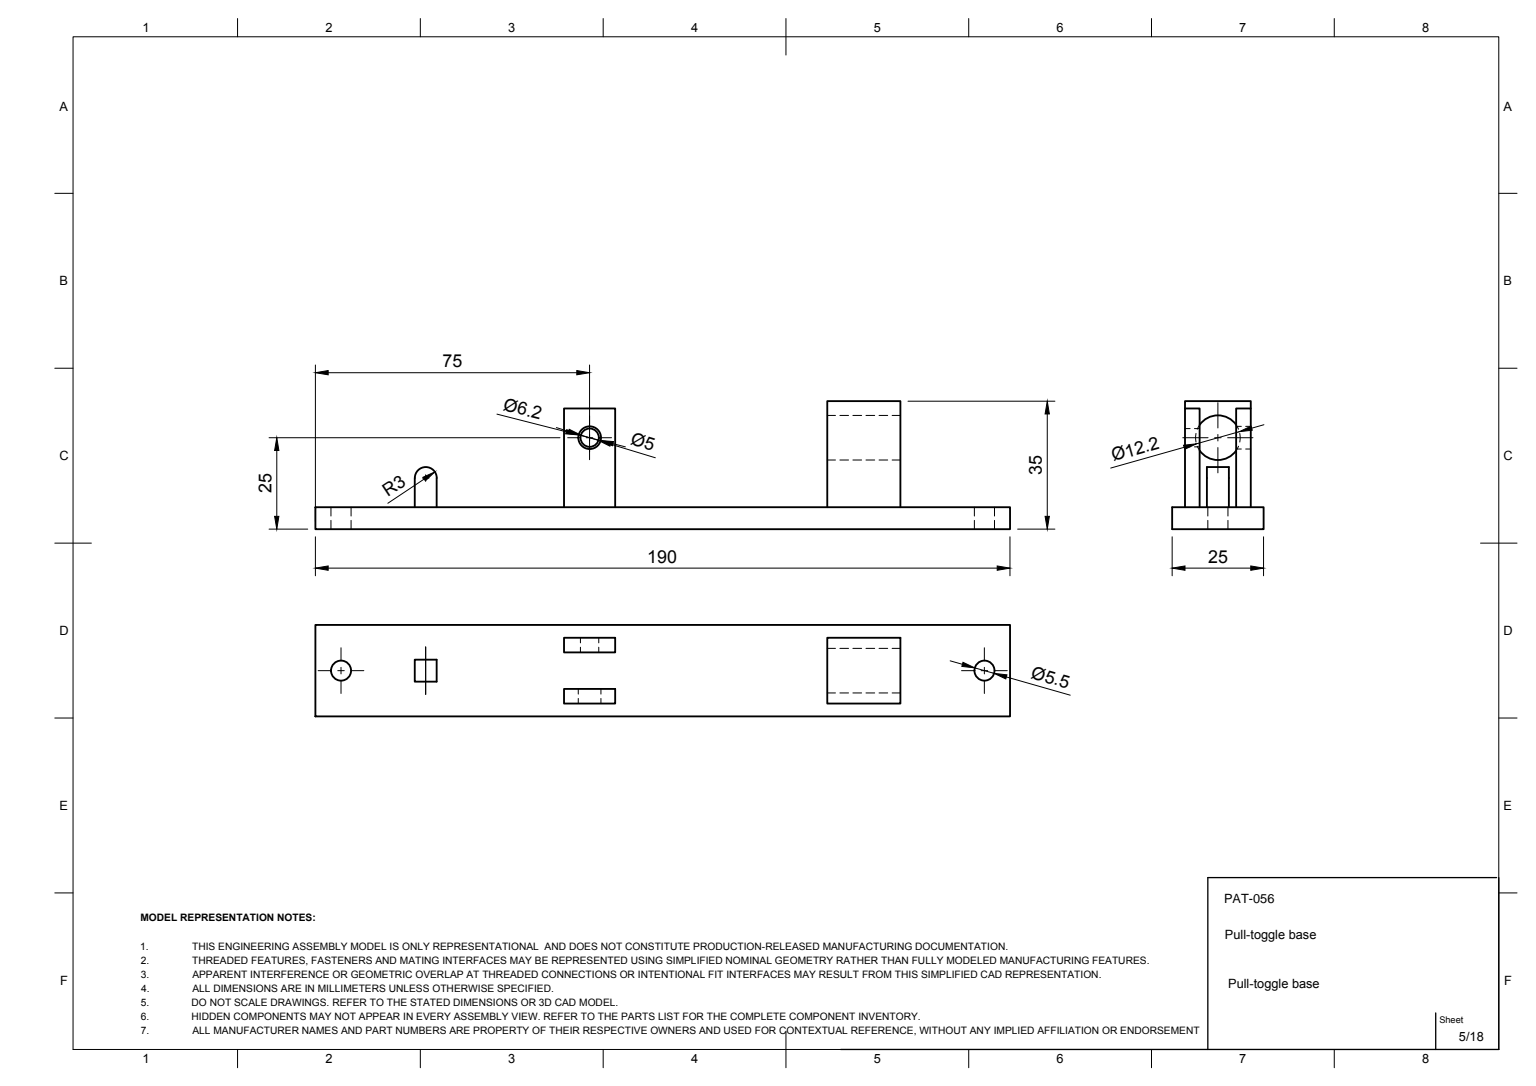
ISO-10303-21;
HEADER;
/* Generated by software containing ST-Developer
 * from STEP Tools, Inc. (www.steptools.com) 
 */

FILE_DESCRIPTION(
/* description */ ('Hook toggle clamp'),
/* implementation_level */ '2;1');

FILE_NAME(
/* name */ 'Pull-toggle base.step',
/* time_stamp */ '2026-10-27T21:56:56-07:00',
/* author */ (''),
/* organization */ (''),
/* preprocessor_version */ 'ST-DEVELOPER v20.2',
/* originating_system */ 'Autodesk Translation Framework v15.17.0.0',
/* authorisation */ '');

FILE_SCHEMA (('AUTOMOTIVE_DESIGN { 1 0 10303 214 3 1 1 }'));
ENDSEC;

DATA;
#10=MECHANICAL_DESIGN_GEOMETRIC_PRESENTATION_REPRESENTATION('',(#189),#5458);
#155=SHAPE_REPRESENTATION_RELATIONSHIP('SRR','None',#5536,#172);
#172=ADVANCED_BREP_SHAPE_REPRESENTATION('',(#206),#5438);
#189=STYLED_ITEM('',(#5696),#206);
#206=MANIFOLD_SOLID_BREP('Body1',#2970);
#222=FACE_BOUND('',#577,.T.);
#223=FACE_BOUND('',#579,.T.);
#224=FACE_BOUND('',#584,.T.);
#225=FACE_BOUND('',#589,.T.);
#226=FACE_BOUND('',#591,.T.);
#227=FACE_BOUND('',#596,.T.);
#228=FACE_BOUND('',#602,.T.);
#229=FACE_BOUND('',#603,.T.);
#230=FACE_BOUND('',#604,.T.);
#231=FACE_BOUND('',#605,.T.);
#232=FACE_BOUND('',#606,.T.);
#233=FACE_BOUND('',#607,.T.);
#234=FACE_BOUND('',#609,.T.);
#235=FACE_BOUND('',#610,.T.);
#278=PLANE('',#3182);
#279=PLANE('',#3183);
#280=PLANE('',#3184);
#281=PLANE('',#3188);
#282=PLANE('',#3198);
#283=PLANE('',#3199);
#284=PLANE('',#3200);
#285=PLANE('',#3201);
#286=PLANE('',#3202);
#287=PLANE('',#3206);
#288=PLANE('',#3207);
#289=PLANE('',#3208);
#290=PLANE('',#3209);
#291=PLANE('',#3210);
#292=PLANE('',#3211);
#293=PLANE('',#3212);
#294=PLANE('',#3213);
#295=PLANE('',#3214);
#296=PLANE('',#3215);
#297=PLANE('',#3216);
#298=PLANE('',#3217);
#299=PLANE('',#3218);
#300=PLANE('',#3219);
#301=PLANE('',#3220);
#302=PLANE('',#3221);
#393=FACE_OUTER_BOUND('',#566,.T.);
#394=FACE_OUTER_BOUND('',#567,.T.);
#395=FACE_OUTER_BOUND('',#568,.T.);
#396=FACE_OUTER_BOUND('',#569,.T.);
#397=FACE_OUTER_BOUND('',#570,.T.);
#398=FACE_OUTER_BOUND('',#571,.T.);
#399=FACE_OUTER_BOUND('',#572,.T.);
#400=FACE_OUTER_BOUND('',#573,.T.);
#401=FACE_OUTER_BOUND('',#574,.T.);
#402=FACE_OUTER_BOUND('',#575,.T.);
#403=FACE_OUTER_BOUND('',#576,.T.);
#404=FACE_OUTER_BOUND('',#578,.T.);
#405=FACE_OUTER_BOUND('',#580,.T.);
#406=FACE_OUTER_BOUND('',#581,.T.);
#407=FACE_OUTER_BOUND('',#582,.T.);
#408=FACE_OUTER_BOUND('',#583,.T.);
#409=FACE_OUTER_BOUND('',#585,.T.);
#410=FACE_OUTER_BOUND('',#586,.T.);
#411=FACE_OUTER_BOUND('',#587,.T.);
#412=FACE_OUTER_BOUND('',#588,.T.);
#413=FACE_OUTER_BOUND('',#590,.T.);
#414=FACE_OUTER_BOUND('',#592,.T.);
#415=FACE_OUTER_BOUND('',#593,.T.);
#416=FACE_OUTER_BOUND('',#594,.T.);
#417=FACE_OUTER_BOUND('',#595,.T.);
#418=FACE_OUTER_BOUND('',#597,.T.);
#419=FACE_OUTER_BOUND('',#598,.T.);
#420=FACE_OUTER_BOUND('',#599,.T.);
#421=FACE_OUTER_BOUND('',#600,.T.);
#422=FACE_OUTER_BOUND('',#601,.T.);
#423=FACE_OUTER_BOUND('',#608,.T.);
#566=EDGE_LOOP('',(#2001,#2002,#2003,#2004));
#567=EDGE_LOOP('',(#2005,#2006,#2007,#2008));
#568=EDGE_LOOP('',(#2009,#2010,#2011,#2012));
#569=EDGE_LOOP('',(#2013,#2014,#2015,#2016));
#570=EDGE_LOOP('',(#2017,#2018,#2019,#2020));
#571=EDGE_LOOP('',(#2021,#2022,#2023,#2024));
#572=EDGE_LOOP('',(#2025,#2026,#2027,#2028));
#573=EDGE_LOOP('',(#2029,#2030,#2031,#2032));
#574=EDGE_LOOP('',(#2033,#2034,#2035,#2036));
#575=EDGE_LOOP('',(#2037,#2038,#2039,#2040));
#576=EDGE_LOOP('',(#2041,#2042,#2043,#2044));
#577=EDGE_LOOP('',(#2045));
#578=EDGE_LOOP('',(#2046,#2047,#2048,#2049));
#579=EDGE_LOOP('',(#2050));
#580=EDGE_LOOP('',(#2051,#2052,#2053,#2054));
#581=EDGE_LOOP('',(#2055,#2056,#2057,#2058));
#582=EDGE_LOOP('',(#2059,#2060,#2061,#2062));
#583=EDGE_LOOP('',(#2063,#2064,#2065,#2066));
#584=EDGE_LOOP('',(#2067));
#585=EDGE_LOOP('',(#2068,#2069,#2070,#2071));
#586=EDGE_LOOP('',(#2072,#2073,#2074,#2075));
#587=EDGE_LOOP('',(#2076,#2077,#2078,#2079));
#588=EDGE_LOOP('',(#2080,#2081,#2082,#2083));
#589=EDGE_LOOP('',(#2084));
#590=EDGE_LOOP('',(#2085,#2086,#2087,#2088));
#591=EDGE_LOOP('',(#2089));
#592=EDGE_LOOP('',(#2090,#2091,#2092,#2093));
#593=EDGE_LOOP('',(#2094,#2095,#2096,#2097));
#594=EDGE_LOOP('',(#2098,#2099,#2100,#2101));
#595=EDGE_LOOP('',(#2102,#2103,#2104,#2105));
#596=EDGE_LOOP('',(#2106));
#597=EDGE_LOOP('',(#2107,#2108,#2109,#2110));
#598=EDGE_LOOP('',(#2111,#2112,#2113,#2114));
#599=EDGE_LOOP('',(#2115,#2116,#2117,#2118));
#600=EDGE_LOOP('',(#2119,#2120,#2121,#2122));
#601=EDGE_LOOP('',(#2123,#2124,#2125,#2126));
#602=EDGE_LOOP('',(#2127,#2128,#2129,#2130));
#603=EDGE_LOOP('',(#2131));
#604=EDGE_LOOP('',(#2132));
#605=EDGE_LOOP('',(#2133,#2134,#2135,#2136));
#606=EDGE_LOOP('',(#2137,#2138,#2139,#2140));
#607=EDGE_LOOP('',(#2141,#2142,#2143,#2144));
#608=EDGE_LOOP('',(#2145,#2146,#2147,#2148));
#609=EDGE_LOOP('',(#2149));
#610=EDGE_LOOP('',(#2150));
#795=LINE('',#4425,#1032);
#796=LINE('',#4430,#1033);
#797=LINE('',#4432,#1034);
#798=LINE('',#4434,#1035);
#799=LINE('',#4435,#1036);
#800=LINE('',#4439,#1037);
#801=LINE('',#4441,#1038);
#802=LINE('',#4443,#1039);
#803=LINE('',#4444,#1040);
#804=LINE('',#4447,#1041);
#805=LINE('',#4451,#1042);
#806=LINE('',#4456,#1043);
#807=LINE('',#4462,#1044);
#808=LINE('',#4468,#1045);
#809=LINE('',#4473,#1046);
#810=LINE('',#4475,#1047);
#811=LINE('',#4477,#1048);
#812=LINE('',#4478,#1049);
#813=LINE('',#4481,#1050);
#814=LINE('',#4483,#1051);
#815=LINE('',#4484,#1052);
#816=LINE('',#4487,#1053);
#817=LINE('',#4489,#1054);
#818=LINE('',#4490,#1055);
#819=LINE('',#4492,#1056);
#820=LINE('',#4494,#1057);
#821=LINE('',#4499,#1058);
#822=LINE('',#4504,#1059);
#823=LINE('',#4506,#1060);
#824=LINE('',#4508,#1061);
#825=LINE('',#4509,#1062);
#826=LINE('',#4512,#1063);
#827=LINE('',#4514,#1064);
#828=LINE('',#4515,#1065);
#829=LINE('',#4518,#1066);
#830=LINE('',#4520,#1067);
#831=LINE('',#4521,#1068);
#832=LINE('',#4523,#1069);
#833=LINE('',#4525,#1070);
#834=LINE('',#4529,#1071);
#835=LINE('',#4531,#1072);
#836=LINE('',#4533,#1073);
#837=LINE('',#4534,#1074);
#838=LINE('',#4537,#1075);
#839=LINE('',#4539,#1076);
#840=LINE('',#4540,#1077);
#841=LINE('',#4543,#1078);
#842=LINE('',#4545,#1079);
#843=LINE('',#4546,#1080);
#844=LINE('',#4548,#1081);
#845=LINE('',#4550,#1082);
#846=LINE('',#4554,#1083);
#847=LINE('',#4556,#1084);
#848=LINE('',#4558,#1085);
#849=LINE('',#4559,#1086);
#850=LINE('',#4562,#1087);
#851=LINE('',#4564,#1088);
#852=LINE('',#4565,#1089);
#853=LINE('',#4568,#1090);
#854=LINE('',#4570,#1091);
#855=LINE('',#4571,#1092);
#856=LINE('',#4573,#1093);
#857=LINE('',#4574,#1094);
#1032=VECTOR('',#3521,0.25);
#1033=VECTOR('',#3526,1.);
#1034=VECTOR('',#3527,1.);
#1035=VECTOR('',#3528,1.);
#1036=VECTOR('',#3529,1.);
#1037=VECTOR('',#3532,1.);
#1038=VECTOR('',#3533,1.);
#1039=VECTOR('',#3534,1.);
#1040=VECTOR('',#3535,1.);
#1041=VECTOR('',#3540,1.);
#1042=VECTOR('',#3547,1.);
#1043=VECTOR('',#3552,0.275);
#1044=VECTOR('',#3559,0.275);
#1045=VECTOR('',#3566,0.61);
#1046=VECTOR('',#3571,1.);
#1047=VECTOR('',#3572,1.);
#1048=VECTOR('',#3573,1.);
#1049=VECTOR('',#3574,1.);
#1050=VECTOR('',#3577,1.);
#1051=VECTOR('',#3578,1.);
#1052=VECTOR('',#3579,1.);
#1053=VECTOR('',#3582,1.);
#1054=VECTOR('',#3583,1.);
#1055=VECTOR('',#3584,1.);
#1056=VECTOR('',#3587,1.);
#1057=VECTOR('',#3590,1.);
#1058=VECTOR('',#3595,0.31);
#1059=VECTOR('',#3600,1.);
#1060=VECTOR('',#3601,1.);
#1061=VECTOR('',#3602,1.);
#1062=VECTOR('',#3603,1.);
#1063=VECTOR('',#3606,1.);
#1064=VECTOR('',#3607,1.);
#1065=VECTOR('',#3608,1.);
#1066=VECTOR('',#3611,1.);
#1067=VECTOR('',#3612,1.);
#1068=VECTOR('',#3613,1.);
#1069=VECTOR('',#3616,1.);
#1070=VECTOR('',#3619,1.);
#1071=VECTOR('',#3622,1.);
#1072=VECTOR('',#3623,1.);
#1073=VECTOR('',#3624,1.);
#1074=VECTOR('',#3625,1.);
#1075=VECTOR('',#3628,1.);
#1076=VECTOR('',#3629,1.);
#1077=VECTOR('',#3630,1.);
#1078=VECTOR('',#3633,1.);
#1079=VECTOR('',#3634,1.);
#1080=VECTOR('',#3635,1.);
#1081=VECTOR('',#3638,1.);
#1082=VECTOR('',#3641,1.);
#1083=VECTOR('',#3644,1.);
#1084=VECTOR('',#3645,1.);
#1085=VECTOR('',#3646,1.);
#1086=VECTOR('',#3647,1.);
#1087=VECTOR('',#3650,1.);
#1088=VECTOR('',#3651,1.);
#1089=VECTOR('',#3652,1.);
#1090=VECTOR('',#3655,1.);
#1091=VECTOR('',#3656,1.);
#1092=VECTOR('',#3657,1.);
#1093=VECTOR('',#3660,1.);
#1094=VECTOR('',#3661,1.);
#1269=CIRCLE('',#3180,0.25);
#1270=CIRCLE('',#3181,0.25);
#1271=CIRCLE('',#3185,0.3);
#1272=CIRCLE('',#3187,0.3);
#1273=CIRCLE('',#3190,0.275);
#1274=CIRCLE('',#3191,0.275);
#1275=CIRCLE('',#3193,0.275);
#1276=CIRCLE('',#3194,0.275);
#1277=CIRCLE('',#3196,0.61);
#1278=CIRCLE('',#3197,0.61);
#1279=CIRCLE('',#3204,0.31);
#1280=CIRCLE('',#3205,0.31);
#1382=VERTEX_POINT('',#4422);
#1383=VERTEX_POINT('',#4424);
#1384=VERTEX_POINT('',#4428);
#1385=VERTEX_POINT('',#4429);
#1386=VERTEX_POINT('',#4431);
#1387=VERTEX_POINT('',#4433);
#1388=VERTEX_POINT('',#4437);
#1389=VERTEX_POINT('',#4438);
#1390=VERTEX_POINT('',#4440);
#1391=VERTEX_POINT('',#4442);
#1392=VERTEX_POINT('',#4453);
#1393=VERTEX_POINT('',#4455);
#1394=VERTEX_POINT('',#4459);
#1395=VERTEX_POINT('',#4461);
#1396=VERTEX_POINT('',#4465);
#1397=VERTEX_POINT('',#4467);
#1398=VERTEX_POINT('',#4471);
#1399=VERTEX_POINT('',#4472);
#1400=VERTEX_POINT('',#4474);
#1401=VERTEX_POINT('',#4476);
#1402=VERTEX_POINT('',#4480);
#1403=VERTEX_POINT('',#4482);
#1404=VERTEX_POINT('',#4486);
#1405=VERTEX_POINT('',#4488);
#1406=VERTEX_POINT('',#4496);
#1407=VERTEX_POINT('',#4498);
#1408=VERTEX_POINT('',#4502);
#1409=VERTEX_POINT('',#4503);
#1410=VERTEX_POINT('',#4505);
#1411=VERTEX_POINT('',#4507);
#1412=VERTEX_POINT('',#4511);
#1413=VERTEX_POINT('',#4513);
#1414=VERTEX_POINT('',#4517);
#1415=VERTEX_POINT('',#4519);
#1416=VERTEX_POINT('',#4527);
#1417=VERTEX_POINT('',#4528);
#1418=VERTEX_POINT('',#4530);
#1419=VERTEX_POINT('',#4532);
#1420=VERTEX_POINT('',#4536);
#1421=VERTEX_POINT('',#4538);
#1422=VERTEX_POINT('',#4542);
#1423=VERTEX_POINT('',#4544);
#1424=VERTEX_POINT('',#4552);
#1425=VERTEX_POINT('',#4553);
#1426=VERTEX_POINT('',#4555);
#1427=VERTEX_POINT('',#4557);
#1428=VERTEX_POINT('',#4561);
#1429=VERTEX_POINT('',#4563);
#1430=VERTEX_POINT('',#4567);
#1431=VERTEX_POINT('',#4569);
#1627=EDGE_CURVE('',#1382,#1382,#1269,.T.);
#1628=EDGE_CURVE('',#1382,#1383,#795,.T.);
#1629=EDGE_CURVE('',#1383,#1383,#1270,.T.);
#1630=EDGE_CURVE('',#1384,#1385,#796,.T.);
#1631=EDGE_CURVE('',#1386,#1384,#797,.T.);
#1632=EDGE_CURVE('',#1387,#1386,#798,.T.);
#1633=EDGE_CURVE('',#1385,#1387,#799,.T.);
#1634=EDGE_CURVE('',#1388,#1389,#800,.T.);
#1635=EDGE_CURVE('',#1390,#1388,#801,.T.);
#1636=EDGE_CURVE('',#1390,#1391,#802,.T.);
#1637=EDGE_CURVE('',#1389,#1391,#803,.T.);
#1638=EDGE_CURVE('',#1390,#1387,#1271,.T.);
#1639=EDGE_CURVE('',#1385,#1388,#804,.T.);
#1640=EDGE_CURVE('',#1391,#1386,#1272,.T.);
#1641=EDGE_CURVE('',#1389,#1384,#805,.T.);
#1642=EDGE_CURVE('',#1392,#1392,#1273,.T.);
#1643=EDGE_CURVE('',#1392,#1393,#806,.T.);
#1644=EDGE_CURVE('',#1393,#1393,#1274,.T.);
#1645=EDGE_CURVE('',#1394,#1394,#1275,.T.);
#1646=EDGE_CURVE('',#1394,#1395,#807,.T.);
#1647=EDGE_CURVE('',#1395,#1395,#1276,.T.);
#1648=EDGE_CURVE('',#1396,#1396,#1277,.T.);
#1649=EDGE_CURVE('',#1396,#1397,#808,.T.);
#1650=EDGE_CURVE('',#1397,#1397,#1278,.T.);
#1651=EDGE_CURVE('',#1398,#1399,#809,.T.);
#1652=EDGE_CURVE('',#1398,#1400,#810,.T.);
#1653=EDGE_CURVE('',#1400,#1401,#811,.T.);
#1654=EDGE_CURVE('',#1401,#1399,#812,.T.);
#1655=EDGE_CURVE('',#1402,#1398,#813,.T.);
#1656=EDGE_CURVE('',#1403,#1402,#814,.T.);
#1657=EDGE_CURVE('',#1400,#1403,#815,.T.);
#1658=EDGE_CURVE('',#1399,#1404,#816,.T.);
#1659=EDGE_CURVE('',#1401,#1405,#817,.T.);
#1660=EDGE_CURVE('',#1404,#1405,#818,.T.);
#1661=EDGE_CURVE('',#1405,#1403,#819,.T.);
#1662=EDGE_CURVE('',#1404,#1402,#820,.T.);
#1663=EDGE_CURVE('',#1406,#1406,#1279,.T.);
#1664=EDGE_CURVE('',#1406,#1407,#821,.T.);
#1665=EDGE_CURVE('',#1407,#1407,#1280,.T.);
#1666=EDGE_CURVE('',#1408,#1409,#822,.T.);
#1667=EDGE_CURVE('',#1408,#1410,#823,.T.);
#1668=EDGE_CURVE('',#1410,#1411,#824,.T.);
#1669=EDGE_CURVE('',#1411,#1409,#825,.T.);
#1670=EDGE_CURVE('',#1412,#1408,#826,.T.);
#1671=EDGE_CURVE('',#1413,#1412,#827,.T.);
#1672=EDGE_CURVE('',#1410,#1413,#828,.T.);
#1673=EDGE_CURVE('',#1409,#1414,#829,.T.);
#1674=EDGE_CURVE('',#1411,#1415,#830,.T.);
#1675=EDGE_CURVE('',#1414,#1415,#831,.T.);
#1676=EDGE_CURVE('',#1415,#1413,#832,.T.);
#1677=EDGE_CURVE('',#1414,#1412,#833,.T.);
#1678=EDGE_CURVE('',#1416,#1417,#834,.T.);
#1679=EDGE_CURVE('',#1416,#1418,#835,.T.);
#1680=EDGE_CURVE('',#1418,#1419,#836,.T.);
#1681=EDGE_CURVE('',#1419,#1417,#837,.T.);
#1682=EDGE_CURVE('',#1420,#1416,#838,.T.);
#1683=EDGE_CURVE('',#1421,#1420,#839,.T.);
#1684=EDGE_CURVE('',#1418,#1421,#840,.T.);
#1685=EDGE_CURVE('',#1417,#1422,#841,.T.);
#1686=EDGE_CURVE('',#1419,#1423,#842,.T.);
#1687=EDGE_CURVE('',#1422,#1423,#843,.T.);
#1688=EDGE_CURVE('',#1423,#1421,#844,.T.);
#1689=EDGE_CURVE('',#1422,#1420,#845,.T.);
#1690=EDGE_CURVE('',#1424,#1425,#846,.T.);
#1691=EDGE_CURVE('',#1425,#1426,#847,.T.);
#1692=EDGE_CURVE('',#1427,#1426,#848,.T.);
#1693=EDGE_CURVE('',#1424,#1427,#849,.T.);
#1694=EDGE_CURVE('',#1428,#1424,#850,.T.);
#1695=EDGE_CURVE('',#1429,#1427,#851,.T.);
#1696=EDGE_CURVE('',#1428,#1429,#852,.T.);
#1697=EDGE_CURVE('',#1430,#1428,#853,.T.);
#1698=EDGE_CURVE('',#1431,#1429,#854,.T.);
#1699=EDGE_CURVE('',#1430,#1431,#855,.T.);
#1700=EDGE_CURVE('',#1425,#1430,#856,.T.);
#1701=EDGE_CURVE('',#1426,#1431,#857,.T.);
#2001=ORIENTED_EDGE('',*,*,#1627,.F.);
#2002=ORIENTED_EDGE('',*,*,#1628,.T.);
#2003=ORIENTED_EDGE('',*,*,#1629,.T.);
#2004=ORIENTED_EDGE('',*,*,#1628,.F.);
#2005=ORIENTED_EDGE('',*,*,#1630,.F.);
#2006=ORIENTED_EDGE('',*,*,#1631,.F.);
#2007=ORIENTED_EDGE('',*,*,#1632,.F.);
#2008=ORIENTED_EDGE('',*,*,#1633,.F.);
#2009=ORIENTED_EDGE('',*,*,#1634,.F.);
#2010=ORIENTED_EDGE('',*,*,#1635,.F.);
#2011=ORIENTED_EDGE('',*,*,#1636,.T.);
#2012=ORIENTED_EDGE('',*,*,#1637,.F.);
#2013=ORIENTED_EDGE('',*,*,#1638,.F.);
#2014=ORIENTED_EDGE('',*,*,#1635,.T.);
#2015=ORIENTED_EDGE('',*,*,#1639,.F.);
#2016=ORIENTED_EDGE('',*,*,#1633,.T.);
#2017=ORIENTED_EDGE('',*,*,#1636,.F.);
#2018=ORIENTED_EDGE('',*,*,#1638,.T.);
#2019=ORIENTED_EDGE('',*,*,#1632,.T.);
#2020=ORIENTED_EDGE('',*,*,#1640,.F.);
#2021=ORIENTED_EDGE('',*,*,#1640,.T.);
#2022=ORIENTED_EDGE('',*,*,#1631,.T.);
#2023=ORIENTED_EDGE('',*,*,#1641,.F.);
#2024=ORIENTED_EDGE('',*,*,#1637,.T.);
#2025=ORIENTED_EDGE('',*,*,#1642,.F.);
#2026=ORIENTED_EDGE('',*,*,#1643,.T.);
#2027=ORIENTED_EDGE('',*,*,#1644,.F.);
#2028=ORIENTED_EDGE('',*,*,#1643,.F.);
#2029=ORIENTED_EDGE('',*,*,#1645,.F.);
#2030=ORIENTED_EDGE('',*,*,#1646,.T.);
#2031=ORIENTED_EDGE('',*,*,#1647,.F.);
#2032=ORIENTED_EDGE('',*,*,#1646,.F.);
#2033=ORIENTED_EDGE('',*,*,#1648,.F.);
#2034=ORIENTED_EDGE('',*,*,#1649,.T.);
#2035=ORIENTED_EDGE('',*,*,#1650,.F.);
#2036=ORIENTED_EDGE('',*,*,#1649,.F.);
#2037=ORIENTED_EDGE('',*,*,#1651,.F.);
#2038=ORIENTED_EDGE('',*,*,#1652,.T.);
#2039=ORIENTED_EDGE('',*,*,#1653,.T.);
#2040=ORIENTED_EDGE('',*,*,#1654,.T.);
#2041=ORIENTED_EDGE('',*,*,#1655,.F.);
#2042=ORIENTED_EDGE('',*,*,#1656,.F.);
#2043=ORIENTED_EDGE('',*,*,#1657,.F.);
#2044=ORIENTED_EDGE('',*,*,#1652,.F.);
#2045=ORIENTED_EDGE('',*,*,#1650,.T.);
#2046=ORIENTED_EDGE('',*,*,#1658,.F.);
#2047=ORIENTED_EDGE('',*,*,#1654,.F.);
#2048=ORIENTED_EDGE('',*,*,#1659,.T.);
#2049=ORIENTED_EDGE('',*,*,#1660,.F.);
#2050=ORIENTED_EDGE('',*,*,#1648,.T.);
#2051=ORIENTED_EDGE('',*,*,#1653,.F.);
#2052=ORIENTED_EDGE('',*,*,#1657,.T.);
#2053=ORIENTED_EDGE('',*,*,#1661,.F.);
#2054=ORIENTED_EDGE('',*,*,#1659,.F.);
#2055=ORIENTED_EDGE('',*,*,#1662,.F.);
#2056=ORIENTED_EDGE('',*,*,#1660,.T.);
#2057=ORIENTED_EDGE('',*,*,#1661,.T.);
#2058=ORIENTED_EDGE('',*,*,#1656,.T.);
#2059=ORIENTED_EDGE('',*,*,#1663,.F.);
#2060=ORIENTED_EDGE('',*,*,#1664,.T.);
#2061=ORIENTED_EDGE('',*,*,#1665,.F.);
#2062=ORIENTED_EDGE('',*,*,#1664,.F.);
#2063=ORIENTED_EDGE('',*,*,#1666,.F.);
#2064=ORIENTED_EDGE('',*,*,#1667,.T.);
#2065=ORIENTED_EDGE('',*,*,#1668,.T.);
#2066=ORIENTED_EDGE('',*,*,#1669,.T.);
#2067=ORIENTED_EDGE('',*,*,#1629,.F.);
#2068=ORIENTED_EDGE('',*,*,#1670,.F.);
#2069=ORIENTED_EDGE('',*,*,#1671,.F.);
#2070=ORIENTED_EDGE('',*,*,#1672,.F.);
#2071=ORIENTED_EDGE('',*,*,#1667,.F.);
#2072=ORIENTED_EDGE('',*,*,#1673,.F.);
#2073=ORIENTED_EDGE('',*,*,#1669,.F.);
#2074=ORIENTED_EDGE('',*,*,#1674,.T.);
#2075=ORIENTED_EDGE('',*,*,#1675,.F.);
#2076=ORIENTED_EDGE('',*,*,#1668,.F.);
#2077=ORIENTED_EDGE('',*,*,#1672,.T.);
#2078=ORIENTED_EDGE('',*,*,#1676,.F.);
#2079=ORIENTED_EDGE('',*,*,#1674,.F.);
#2080=ORIENTED_EDGE('',*,*,#1677,.F.);
#2081=ORIENTED_EDGE('',*,*,#1675,.T.);
#2082=ORIENTED_EDGE('',*,*,#1676,.T.);
#2083=ORIENTED_EDGE('',*,*,#1671,.T.);
#2084=ORIENTED_EDGE('',*,*,#1627,.T.);
#2085=ORIENTED_EDGE('',*,*,#1678,.F.);
#2086=ORIENTED_EDGE('',*,*,#1679,.T.);
#2087=ORIENTED_EDGE('',*,*,#1680,.T.);
#2088=ORIENTED_EDGE('',*,*,#1681,.T.);
#2089=ORIENTED_EDGE('',*,*,#1663,.T.);
#2090=ORIENTED_EDGE('',*,*,#1682,.F.);
#2091=ORIENTED_EDGE('',*,*,#1683,.F.);
#2092=ORIENTED_EDGE('',*,*,#1684,.F.);
#2093=ORIENTED_EDGE('',*,*,#1679,.F.);
#2094=ORIENTED_EDGE('',*,*,#1685,.F.);
#2095=ORIENTED_EDGE('',*,*,#1681,.F.);
#2096=ORIENTED_EDGE('',*,*,#1686,.T.);
#2097=ORIENTED_EDGE('',*,*,#1687,.F.);
#2098=ORIENTED_EDGE('',*,*,#1680,.F.);
#2099=ORIENTED_EDGE('',*,*,#1684,.T.);
#2100=ORIENTED_EDGE('',*,*,#1688,.F.);
#2101=ORIENTED_EDGE('',*,*,#1686,.F.);
#2102=ORIENTED_EDGE('',*,*,#1689,.F.);
#2103=ORIENTED_EDGE('',*,*,#1687,.T.);
#2104=ORIENTED_EDGE('',*,*,#1688,.T.);
#2105=ORIENTED_EDGE('',*,*,#1683,.T.);
#2106=ORIENTED_EDGE('',*,*,#1665,.T.);
#2107=ORIENTED_EDGE('',*,*,#1690,.T.);
#2108=ORIENTED_EDGE('',*,*,#1691,.T.);
#2109=ORIENTED_EDGE('',*,*,#1692,.F.);
#2110=ORIENTED_EDGE('',*,*,#1693,.F.);
#2111=ORIENTED_EDGE('',*,*,#1694,.T.);
#2112=ORIENTED_EDGE('',*,*,#1693,.T.);
#2113=ORIENTED_EDGE('',*,*,#1695,.F.);
#2114=ORIENTED_EDGE('',*,*,#1696,.F.);
#2115=ORIENTED_EDGE('',*,*,#1697,.T.);
#2116=ORIENTED_EDGE('',*,*,#1696,.T.);
#2117=ORIENTED_EDGE('',*,*,#1698,.F.);
#2118=ORIENTED_EDGE('',*,*,#1699,.F.);
#2119=ORIENTED_EDGE('',*,*,#1700,.T.);
#2120=ORIENTED_EDGE('',*,*,#1699,.T.);
#2121=ORIENTED_EDGE('',*,*,#1701,.F.);
#2122=ORIENTED_EDGE('',*,*,#1691,.F.);
#2123=ORIENTED_EDGE('',*,*,#1701,.T.);
#2124=ORIENTED_EDGE('',*,*,#1698,.T.);
#2125=ORIENTED_EDGE('',*,*,#1695,.T.);
#2126=ORIENTED_EDGE('',*,*,#1692,.T.);
#2127=ORIENTED_EDGE('',*,*,#1630,.T.);
#2128=ORIENTED_EDGE('',*,*,#1639,.T.);
#2129=ORIENTED_EDGE('',*,*,#1634,.T.);
#2130=ORIENTED_EDGE('',*,*,#1641,.T.);
#2131=ORIENTED_EDGE('',*,*,#1644,.T.);
#2132=ORIENTED_EDGE('',*,*,#1647,.T.);
#2133=ORIENTED_EDGE('',*,*,#1655,.T.);
#2134=ORIENTED_EDGE('',*,*,#1651,.T.);
#2135=ORIENTED_EDGE('',*,*,#1658,.T.);
#2136=ORIENTED_EDGE('',*,*,#1662,.T.);
#2137=ORIENTED_EDGE('',*,*,#1670,.T.);
#2138=ORIENTED_EDGE('',*,*,#1666,.T.);
#2139=ORIENTED_EDGE('',*,*,#1673,.T.);
#2140=ORIENTED_EDGE('',*,*,#1677,.T.);
#2141=ORIENTED_EDGE('',*,*,#1682,.T.);
#2142=ORIENTED_EDGE('',*,*,#1678,.T.);
#2143=ORIENTED_EDGE('',*,*,#1685,.T.);
#2144=ORIENTED_EDGE('',*,*,#1689,.T.);
#2145=ORIENTED_EDGE('',*,*,#1700,.F.);
#2146=ORIENTED_EDGE('',*,*,#1690,.F.);
#2147=ORIENTED_EDGE('',*,*,#1694,.F.);
#2148=ORIENTED_EDGE('',*,*,#1697,.F.);
#2149=ORIENTED_EDGE('',*,*,#1642,.T.);
#2150=ORIENTED_EDGE('',*,*,#1645,.T.);
#2749=CYLINDRICAL_SURFACE('',#3179,0.25);
#2750=CYLINDRICAL_SURFACE('',#3186,0.3);
#2751=CYLINDRICAL_SURFACE('',#3189,0.275);
#2752=CYLINDRICAL_SURFACE('',#3192,0.275);
#2753=CYLINDRICAL_SURFACE('',#3195,0.61);
#2754=CYLINDRICAL_SURFACE('',#3203,0.31);
#2797=ADVANCED_FACE('',(#393),#2749,.F.);
#2798=ADVANCED_FACE('',(#394),#278,.T.);
#2799=ADVANCED_FACE('',(#395),#279,.T.);
#2800=ADVANCED_FACE('',(#396),#280,.F.);
#2801=ADVANCED_FACE('',(#397),#2750,.T.);
#2802=ADVANCED_FACE('',(#398),#281,.T.);
#2803=ADVANCED_FACE('',(#399),#2751,.F.);
#2804=ADVANCED_FACE('',(#400),#2752,.F.);
#2805=ADVANCED_FACE('',(#401),#2753,.F.);
#2806=ADVANCED_FACE('',(#402),#282,.F.);
#2807=ADVANCED_FACE('',(#403,#222),#283,.T.);
#2808=ADVANCED_FACE('',(#404,#223),#284,.T.);
#2809=ADVANCED_FACE('',(#405),#285,.T.);
#2810=ADVANCED_FACE('',(#406),#286,.T.);
#2811=ADVANCED_FACE('',(#407),#2754,.F.);
#2812=ADVANCED_FACE('',(#408,#224),#287,.F.);
#2813=ADVANCED_FACE('',(#409),#288,.T.);
#2814=ADVANCED_FACE('',(#410),#289,.T.);
#2815=ADVANCED_FACE('',(#411),#290,.T.);
#2816=ADVANCED_FACE('',(#412,#225),#291,.T.);
#2817=ADVANCED_FACE('',(#413,#226),#292,.F.);
#2818=ADVANCED_FACE('',(#414),#293,.T.);
#2819=ADVANCED_FACE('',(#415),#294,.T.);
#2820=ADVANCED_FACE('',(#416),#295,.T.);
#2821=ADVANCED_FACE('',(#417,#227),#296,.T.);
#2822=ADVANCED_FACE('',(#418),#297,.T.);
#2823=ADVANCED_FACE('',(#419),#298,.T.);
#2824=ADVANCED_FACE('',(#420),#299,.T.);
#2825=ADVANCED_FACE('',(#421),#300,.T.);
#2826=ADVANCED_FACE('',(#422,#228,#229,#230,#231,#232,#233),#301,.T.);
#2827=ADVANCED_FACE('',(#423,#234,#235),#302,.F.);
#2970=CLOSED_SHELL('',(#2797,#2798,#2799,#2800,#2801,#2802,#2803,#2804,
#2805,#2806,#2807,#2808,#2809,#2810,#2811,#2812,#2813,#2814,#2815,#2816,
#2817,#2818,#2819,#2820,#2821,#2822,#2823,#2824,#2825,#2826,#2827));
#3178=AXIS2_PLACEMENT_3D('',#4420,#3515,#3516);
#3179=AXIS2_PLACEMENT_3D('',#4421,#3517,#3518);
#3180=AXIS2_PLACEMENT_3D('',#4423,#3519,#3520);
#3181=AXIS2_PLACEMENT_3D('',#4426,#3522,#3523);
#3182=AXIS2_PLACEMENT_3D('',#4427,#3524,#3525);
#3183=AXIS2_PLACEMENT_3D('',#4436,#3530,#3531);
#3184=AXIS2_PLACEMENT_3D('',#4445,#3536,#3537);
#3185=AXIS2_PLACEMENT_3D('',#4446,#3538,#3539);
#3186=AXIS2_PLACEMENT_3D('',#4448,#3541,#3542);
#3187=AXIS2_PLACEMENT_3D('',#4449,#3543,#3544);
#3188=AXIS2_PLACEMENT_3D('',#4450,#3545,#3546);
#3189=AXIS2_PLACEMENT_3D('',#4452,#3548,#3549);
#3190=AXIS2_PLACEMENT_3D('',#4454,#3550,#3551);
#3191=AXIS2_PLACEMENT_3D('',#4457,#3553,#3554);
#3192=AXIS2_PLACEMENT_3D('',#4458,#3555,#3556);
#3193=AXIS2_PLACEMENT_3D('',#4460,#3557,#3558);
#3194=AXIS2_PLACEMENT_3D('',#4463,#3560,#3561);
#3195=AXIS2_PLACEMENT_3D('',#4464,#3562,#3563);
#3196=AXIS2_PLACEMENT_3D('',#4466,#3564,#3565);
#3197=AXIS2_PLACEMENT_3D('',#4469,#3567,#3568);
#3198=AXIS2_PLACEMENT_3D('',#4470,#3569,#3570);
#3199=AXIS2_PLACEMENT_3D('',#4479,#3575,#3576);
#3200=AXIS2_PLACEMENT_3D('',#4485,#3580,#3581);
#3201=AXIS2_PLACEMENT_3D('',#4491,#3585,#3586);
#3202=AXIS2_PLACEMENT_3D('',#4493,#3588,#3589);
#3203=AXIS2_PLACEMENT_3D('',#4495,#3591,#3592);
#3204=AXIS2_PLACEMENT_3D('',#4497,#3593,#3594);
#3205=AXIS2_PLACEMENT_3D('',#4500,#3596,#3597);
#3206=AXIS2_PLACEMENT_3D('',#4501,#3598,#3599);
#3207=AXIS2_PLACEMENT_3D('',#4510,#3604,#3605);
#3208=AXIS2_PLACEMENT_3D('',#4516,#3609,#3610);
#3209=AXIS2_PLACEMENT_3D('',#4522,#3614,#3615);
#3210=AXIS2_PLACEMENT_3D('',#4524,#3617,#3618);
#3211=AXIS2_PLACEMENT_3D('',#4526,#3620,#3621);
#3212=AXIS2_PLACEMENT_3D('',#4535,#3626,#3627);
#3213=AXIS2_PLACEMENT_3D('',#4541,#3631,#3632);
#3214=AXIS2_PLACEMENT_3D('',#4547,#3636,#3637);
#3215=AXIS2_PLACEMENT_3D('',#4549,#3639,#3640);
#3216=AXIS2_PLACEMENT_3D('',#4551,#3642,#3643);
#3217=AXIS2_PLACEMENT_3D('',#4560,#3648,#3649);
#3218=AXIS2_PLACEMENT_3D('',#4566,#3653,#3654);
#3219=AXIS2_PLACEMENT_3D('',#4572,#3658,#3659);
#3220=AXIS2_PLACEMENT_3D('',#4575,#3662,#3663);
#3221=AXIS2_PLACEMENT_3D('',#4576,#3664,#3665);
#3515=DIRECTION('axis',(0.,0.,1.));
#3516=DIRECTION('refdir',(1.,0.,0.));
#3517=DIRECTION('center_axis',(0.,1.,0.));
#3518=DIRECTION('ref_axis',(1.,0.,0.));
#3519=DIRECTION('center_axis',(0.,-1.,0.));
#3520=DIRECTION('ref_axis',(1.,0.,0.));
#3521=DIRECTION('',(0.,-1.,0.));
#3522=DIRECTION('center_axis',(0.,-1.,0.));
#3523=DIRECTION('ref_axis',(1.,0.,0.));
#3524=DIRECTION('center_axis',(1.,0.,0.));
#3525=DIRECTION('ref_axis',(0.,0.,-1.));
#3526=DIRECTION('',(0.,-1.,0.));
#3527=DIRECTION('',(0.,0.,-1.));
#3528=DIRECTION('',(0.,1.,0.));
#3529=DIRECTION('',(0.,0.,1.));
#3530=DIRECTION('center_axis',(-1.,0.,0.));
#3531=DIRECTION('ref_axis',(0.,0.,1.));
#3532=DIRECTION('',(0.,1.,0.));
#3533=DIRECTION('',(0.,0.,-1.));
#3534=DIRECTION('',(0.,1.,0.));
#3535=DIRECTION('',(0.,0.,1.));
#3536=DIRECTION('center_axis',(0.,1.,0.));
#3537=DIRECTION('ref_axis',(1.,0.,0.));
#3538=DIRECTION('center_axis',(0.,1.,0.));
#3539=DIRECTION('ref_axis',(1.,0.,0.));
#3540=DIRECTION('',(-1.,0.,0.));
#3541=DIRECTION('center_axis',(0.,1.,0.));
#3542=DIRECTION('ref_axis',(1.,0.,0.));
#3543=DIRECTION('center_axis',(0.,1.,0.));
#3544=DIRECTION('ref_axis',(1.,0.,0.));
#3545=DIRECTION('center_axis',(0.,1.,0.));
#3546=DIRECTION('ref_axis',(1.,0.,0.));
#3547=DIRECTION('',(1.,0.,0.));
#3548=DIRECTION('center_axis',(0.,0.,1.));
#3549=DIRECTION('ref_axis',(1.,0.,0.));
#3550=DIRECTION('center_axis',(0.,0.,1.));
#3551=DIRECTION('ref_axis',(1.,0.,0.));
#3552=DIRECTION('',(0.,0.,1.));
#3553=DIRECTION('center_axis',(0.,0.,-1.));
#3554=DIRECTION('ref_axis',(1.,0.,0.));
#3555=DIRECTION('center_axis',(0.,0.,1.));
#3556=DIRECTION('ref_axis',(1.,0.,0.));
#3557=DIRECTION('center_axis',(0.,0.,1.));
#3558=DIRECTION('ref_axis',(1.,0.,0.));
#3559=DIRECTION('',(0.,0.,1.));
#3560=DIRECTION('center_axis',(0.,0.,-1.));
#3561=DIRECTION('ref_axis',(1.,0.,0.));
#3562=DIRECTION('center_axis',(1.,0.,0.));
#3563=DIRECTION('ref_axis',(0.,0.,-1.));
#3564=DIRECTION('center_axis',(1.,0.,0.));
#3565=DIRECTION('ref_axis',(0.,0.,-1.));
#3566=DIRECTION('',(1.,0.,0.));
#3567=DIRECTION('center_axis',(-1.,0.,0.));
#3568=DIRECTION('ref_axis',(0.,0.,-1.));
#3569=DIRECTION('center_axis',(0.,1.,0.));
#3570=DIRECTION('ref_axis',(1.,0.,0.));
#3571=DIRECTION('',(-1.,0.,0.));
#3572=DIRECTION('',(0.,0.,1.));
#3573=DIRECTION('',(-1.,0.,0.));
#3574=DIRECTION('',(0.,0.,-1.));
#3575=DIRECTION('center_axis',(1.,0.,0.));
#3576=DIRECTION('ref_axis',(0.,0.,-1.));
#3577=DIRECTION('',(0.,-1.,0.));
#3578=DIRECTION('',(0.,0.,-1.));
#3579=DIRECTION('',(0.,1.,0.));
#3580=DIRECTION('center_axis',(-1.,0.,0.));
#3581=DIRECTION('ref_axis',(0.,0.,1.));
#3582=DIRECTION('',(0.,1.,0.));
#3583=DIRECTION('',(0.,1.,0.));
#3584=DIRECTION('',(0.,0.,1.));
#3585=DIRECTION('center_axis',(0.,0.,1.));
#3586=DIRECTION('ref_axis',(1.,0.,0.));
#3587=DIRECTION('',(1.,0.,0.));
#3588=DIRECTION('center_axis',(0.,1.,0.));
#3589=DIRECTION('ref_axis',(0.,0.,1.));
#3590=DIRECTION('',(1.,0.,0.));
#3591=DIRECTION('center_axis',(0.,1.,0.));
#3592=DIRECTION('ref_axis',(1.,0.,0.));
#3593=DIRECTION('center_axis',(0.,1.,0.));
#3594=DIRECTION('ref_axis',(1.,0.,0.));
#3595=DIRECTION('',(0.,1.,0.));
#3596=DIRECTION('center_axis',(0.,-1.,0.));
#3597=DIRECTION('ref_axis',(1.,0.,0.));
#3598=DIRECTION('center_axis',(0.,1.,0.));
#3599=DIRECTION('ref_axis',(1.,0.,0.));
#3600=DIRECTION('',(-1.,0.,0.));
#3601=DIRECTION('',(0.,0.,1.));
#3602=DIRECTION('',(-1.,0.,0.));
#3603=DIRECTION('',(0.,0.,-1.));
#3604=DIRECTION('center_axis',(1.,0.,0.));
#3605=DIRECTION('ref_axis',(0.,0.,-1.));
#3606=DIRECTION('',(0.,-1.,0.));
#3607=DIRECTION('',(0.,0.,-1.));
#3608=DIRECTION('',(0.,1.,0.));
#3609=DIRECTION('center_axis',(-1.,0.,0.));
#3610=DIRECTION('ref_axis',(0.,0.,1.));
#3611=DIRECTION('',(0.,1.,0.));
#3612=DIRECTION('',(0.,1.,0.));
#3613=DIRECTION('',(0.,0.,1.));
#3614=DIRECTION('center_axis',(0.,0.,1.));
#3615=DIRECTION('ref_axis',(1.,0.,0.));
#3616=DIRECTION('',(1.,0.,0.));
#3617=DIRECTION('center_axis',(0.,1.,0.));
#3618=DIRECTION('ref_axis',(0.,0.,1.));
#3619=DIRECTION('',(1.,0.,0.));
#3620=DIRECTION('center_axis',(0.,1.,0.));
#3621=DIRECTION('ref_axis',(1.,0.,0.));
#3622=DIRECTION('',(-1.,0.,0.));
#3623=DIRECTION('',(0.,0.,1.));
#3624=DIRECTION('',(-1.,0.,0.));
#3625=DIRECTION('',(0.,0.,-1.));
#3626=DIRECTION('center_axis',(1.,0.,0.));
#3627=DIRECTION('ref_axis',(0.,0.,-1.));
#3628=DIRECTION('',(0.,-1.,0.));
#3629=DIRECTION('',(0.,0.,-1.));
#3630=DIRECTION('',(0.,1.,0.));
#3631=DIRECTION('center_axis',(-1.,0.,0.));
#3632=DIRECTION('ref_axis',(0.,0.,1.));
#3633=DIRECTION('',(0.,1.,0.));
#3634=DIRECTION('',(0.,1.,0.));
#3635=DIRECTION('',(0.,0.,1.));
#3636=DIRECTION('center_axis',(0.,0.,1.));
#3637=DIRECTION('ref_axis',(1.,0.,0.));
#3638=DIRECTION('',(1.,0.,0.));
#3639=DIRECTION('center_axis',(0.,1.,0.));
#3640=DIRECTION('ref_axis',(0.,0.,1.));
#3641=DIRECTION('',(1.,0.,0.));
#3642=DIRECTION('center_axis',(0.,1.,0.));
#3643=DIRECTION('ref_axis',(-1.,0.,0.));
#3644=DIRECTION('',(-1.,0.,0.));
#3645=DIRECTION('',(0.,0.,1.));
#3646=DIRECTION('',(-1.,0.,0.));
#3647=DIRECTION('',(0.,0.,1.));
#3648=DIRECTION('center_axis',(1.,0.,0.));
#3649=DIRECTION('ref_axis',(0.,1.,0.));
#3650=DIRECTION('',(0.,1.,0.));
#3651=DIRECTION('',(0.,1.,0.));
#3652=DIRECTION('',(0.,0.,1.));
#3653=DIRECTION('center_axis',(0.,-1.,0.));
#3654=DIRECTION('ref_axis',(1.,0.,0.));
#3655=DIRECTION('',(1.,0.,0.));
#3656=DIRECTION('',(1.,0.,0.));
#3657=DIRECTION('',(0.,0.,1.));
#3658=DIRECTION('center_axis',(-1.,0.,0.));
#3659=DIRECTION('ref_axis',(0.,-1.,0.));
#3660=DIRECTION('',(0.,-1.,0.));
#3661=DIRECTION('',(0.,-1.,0.));
#3662=DIRECTION('center_axis',(0.,0.,1.));
#3663=DIRECTION('ref_axis',(1.,0.,0.));
#3664=DIRECTION('center_axis',(0.,0.,1.));
#3665=DIRECTION('ref_axis',(1.,0.,0.));
#4420=CARTESIAN_POINT('',(0.,0.,0.));
#4421=CARTESIAN_POINT('Origin',(0.,0.5,2.5));
#4422=CARTESIAN_POINT('',(-0.25,0.9,2.5));
#4423=CARTESIAN_POINT('Origin',(0.,0.9,2.5));
#4424=CARTESIAN_POINT('',(-0.25,0.5,2.5));
#4425=CARTESIAN_POINT('',(-0.25,0.5,2.5));
#4426=CARTESIAN_POINT('Origin',(0.,0.5,2.5));
#4427=CARTESIAN_POINT('Origin',(-4.18287614141286,-0.3,1.39779915763554));
#4428=CARTESIAN_POINT('',(-4.18287614141286,0.3,0.6));
#4429=CARTESIAN_POINT('',(-4.18287614141286,-0.3,0.6));
#4430=CARTESIAN_POINT('',(-4.18287614141286,-0.15,0.6));
#4431=CARTESIAN_POINT('',(-4.18287614141286,0.3,1.39779915763554));
#4432=CARTESIAN_POINT('',(-4.18287614141286,0.3,0.5));
#4433=CARTESIAN_POINT('',(-4.18287614141286,-0.3,1.39779915763554));
#4434=CARTESIAN_POINT('',(-4.18287614141286,-0.3,1.39779915763554));
#4435=CARTESIAN_POINT('',(-4.18287614141286,-0.3,0.5));
#4436=CARTESIAN_POINT('Origin',(-4.78287614141285,-0.3,0.5));
#4437=CARTESIAN_POINT('',(-4.78287614141285,-0.3,0.6));
#4438=CARTESIAN_POINT('',(-4.78287614141285,0.3,0.6));
#4439=CARTESIAN_POINT('',(-4.78287614141285,-0.15,0.6));
#4440=CARTESIAN_POINT('',(-4.78287614141285,-0.3,1.39779915763554));
#4441=CARTESIAN_POINT('',(-4.78287614141285,-0.3,1.39779915763554));
#4442=CARTESIAN_POINT('',(-4.78287614141285,0.3,1.39779915763554));
#4443=CARTESIAN_POINT('',(-4.78287614141285,-0.3,1.39779915763554));
#4444=CARTESIAN_POINT('',(-4.78287614141285,0.3,1.39779915763554));
#4445=CARTESIAN_POINT('Origin',(-4.48287614141285,-0.3,1.39779915763554));
#4446=CARTESIAN_POINT('Origin',(-4.48287614141285,-0.3,1.39779915763554));
#4447=CARTESIAN_POINT('',(-1.24143807070643,-0.3,0.6));
#4448=CARTESIAN_POINT('Origin',(-4.48287614141285,-0.3,1.39779915763554));
#4449=CARTESIAN_POINT('Origin',(-4.48287614141285,0.3,1.39779915763554));
#4450=CARTESIAN_POINT('Origin',(-4.48287614141285,0.3,1.39779915763554));
#4451=CARTESIAN_POINT('',(-1.24143807070643,0.3,0.6));
#4452=CARTESIAN_POINT('Origin',(-6.8,0.,-0.1));
#4453=CARTESIAN_POINT('',(-7.075,-3.36777869765523E-17,0.));
#4454=CARTESIAN_POINT('Origin',(-6.8,0.,0.));
#4455=CARTESIAN_POINT('',(-7.075,3.36777869765523E-17,0.6));
#4456=CARTESIAN_POINT('',(-7.075,-3.36777869765523E-17,-0.1));
#4457=CARTESIAN_POINT('Origin',(-6.8,0.,0.6));
#4458=CARTESIAN_POINT('Origin',(10.8,0.,-0.1));
#4459=CARTESIAN_POINT('',(10.525,-3.36777869765523E-17,0.));
#4460=CARTESIAN_POINT('Origin',(10.8,0.,0.));
#4461=CARTESIAN_POINT('',(10.525,3.36777869765523E-17,0.6));
#4462=CARTESIAN_POINT('',(10.525,-3.36777869765523E-17,-0.1));
#4463=CARTESIAN_POINT('Origin',(10.8,0.,0.6));
#4464=CARTESIAN_POINT('Origin',(6.4,0.,2.5));
#4465=CARTESIAN_POINT('',(6.5,-7.47034547479885E-17,3.11));
#4466=CARTESIAN_POINT('Origin',(6.5,0.,2.5));
#4467=CARTESIAN_POINT('',(8.5,7.47034547479885E-17,3.11));
#4468=CARTESIAN_POINT('',(6.4,-7.47034547479885E-17,3.11));
#4469=CARTESIAN_POINT('Origin',(8.5,0.,2.5));
#4470=CARTESIAN_POINT('Origin',(7.5,-0.9,2.));
#4471=CARTESIAN_POINT('',(8.5,-0.9,0.6));
#4472=CARTESIAN_POINT('',(6.5,-0.9,0.6));
#4473=CARTESIAN_POINT('',(4.75,-0.9,0.6));
#4474=CARTESIAN_POINT('',(8.5,-0.9,3.5));
#4475=CARTESIAN_POINT('',(8.5,-0.9,0.5));
#4476=CARTESIAN_POINT('',(6.5,-0.9,3.5));
#4477=CARTESIAN_POINT('',(8.5,-0.9,3.5));
#4478=CARTESIAN_POINT('',(6.5,-0.9,3.5));
#4479=CARTESIAN_POINT('Origin',(8.5,-0.9,3.5));
#4480=CARTESIAN_POINT('',(8.5,0.9,0.6));
#4481=CARTESIAN_POINT('',(8.5,-0.45,0.6));
#4482=CARTESIAN_POINT('',(8.5,0.9,3.5));
#4483=CARTESIAN_POINT('',(8.5,0.9,0.5));
#4484=CARTESIAN_POINT('',(8.5,-0.9,3.5));
#4485=CARTESIAN_POINT('Origin',(6.5,-0.9,0.5));
#4486=CARTESIAN_POINT('',(6.5,0.9,0.6));
#4487=CARTESIAN_POINT('',(6.5,-0.45,0.6));
#4488=CARTESIAN_POINT('',(6.5,0.9,3.5));
#4489=CARTESIAN_POINT('',(6.5,-0.9,3.5));
#4490=CARTESIAN_POINT('',(6.5,0.9,3.5));
#4491=CARTESIAN_POINT('Origin',(6.5,-0.9,3.5));
#4492=CARTESIAN_POINT('',(8.5,0.9,3.5));
#4493=CARTESIAN_POINT('Origin',(7.5,0.9,2.));
#4494=CARTESIAN_POINT('',(4.75,0.9,0.6));
#4495=CARTESIAN_POINT('Origin',(0.,-1.,2.5));
#4496=CARTESIAN_POINT('',(-0.31,-0.9,2.5));
#4497=CARTESIAN_POINT('Origin',(0.,-0.9,2.5));
#4498=CARTESIAN_POINT('',(-0.31,-0.5,2.5));
#4499=CARTESIAN_POINT('',(-0.31,-1.,2.5));
#4500=CARTESIAN_POINT('Origin',(0.,-0.5,2.5));
#4501=CARTESIAN_POINT('Origin',(0.,0.5,1.9));
#4502=CARTESIAN_POINT('',(0.7,0.5,0.6));
#4503=CARTESIAN_POINT('',(-0.7,0.5,0.6));
#4504=CARTESIAN_POINT('',(1.,0.5,0.6));
#4505=CARTESIAN_POINT('',(0.7,0.5,3.3));
#4506=CARTESIAN_POINT('',(0.7,0.5,0.5));
#4507=CARTESIAN_POINT('',(-0.7,0.5,3.3));
#4508=CARTESIAN_POINT('',(0.7,0.5,3.3));
#4509=CARTESIAN_POINT('',(-0.7,0.5,3.3));
#4510=CARTESIAN_POINT('Origin',(0.7,0.5,3.3));
#4511=CARTESIAN_POINT('',(0.7,0.9,0.6));
#4512=CARTESIAN_POINT('',(0.7,0.25,0.6));
#4513=CARTESIAN_POINT('',(0.7,0.9,3.3));
#4514=CARTESIAN_POINT('',(0.7,0.9,0.5));
#4515=CARTESIAN_POINT('',(0.7,0.5,3.3));
#4516=CARTESIAN_POINT('Origin',(-0.7,0.5,0.5));
#4517=CARTESIAN_POINT('',(-0.7,0.9,0.6));
#4518=CARTESIAN_POINT('',(-0.7,0.25,0.6));
#4519=CARTESIAN_POINT('',(-0.7,0.9,3.3));
#4520=CARTESIAN_POINT('',(-0.7,0.5,3.3));
#4521=CARTESIAN_POINT('',(-0.7,0.9,3.3));
#4522=CARTESIAN_POINT('Origin',(-0.7,0.5,3.3));
#4523=CARTESIAN_POINT('',(0.7,0.9,3.3));
#4524=CARTESIAN_POINT('Origin',(0.,0.9,1.9));
#4525=CARTESIAN_POINT('',(1.,0.9,0.6));
#4526=CARTESIAN_POINT('Origin',(0.,-0.9,1.9));
#4527=CARTESIAN_POINT('',(0.7,-0.9,0.6));
#4528=CARTESIAN_POINT('',(-0.7,-0.9,0.6));
#4529=CARTESIAN_POINT('',(1.,-0.9,0.6));
#4530=CARTESIAN_POINT('',(0.7,-0.9,3.3));
#4531=CARTESIAN_POINT('',(0.7,-0.9,0.5));
#4532=CARTESIAN_POINT('',(-0.7,-0.9,3.3));
#4533=CARTESIAN_POINT('',(0.7,-0.9,3.3));
#4534=CARTESIAN_POINT('',(-0.7,-0.9,3.3));
#4535=CARTESIAN_POINT('Origin',(0.7,-0.9,3.3));
#4536=CARTESIAN_POINT('',(0.7,-0.5,0.6));
#4537=CARTESIAN_POINT('',(0.7,-0.45,0.6));
#4538=CARTESIAN_POINT('',(0.7,-0.5,3.3));
#4539=CARTESIAN_POINT('',(0.7,-0.5,0.5));
#4540=CARTESIAN_POINT('',(0.7,-0.9,3.3));
#4541=CARTESIAN_POINT('Origin',(-0.7,-0.9,0.5));
#4542=CARTESIAN_POINT('',(-0.7,-0.5,0.6));
#4543=CARTESIAN_POINT('',(-0.7,-0.45,0.6));
#4544=CARTESIAN_POINT('',(-0.7,-0.5,3.3));
#4545=CARTESIAN_POINT('',(-0.7,-0.9,3.3));
#4546=CARTESIAN_POINT('',(-0.7,-0.5,3.3));
#4547=CARTESIAN_POINT('Origin',(-0.7,-0.9,3.3));
#4548=CARTESIAN_POINT('',(0.7,-0.5,3.3));
#4549=CARTESIAN_POINT('Origin',(0.,-0.5,1.9));
#4550=CARTESIAN_POINT('',(1.,-0.5,0.6));
#4551=CARTESIAN_POINT('Origin',(11.5,1.25,0.));
#4552=CARTESIAN_POINT('',(11.5,1.25,0.));
#4553=CARTESIAN_POINT('',(-7.5,1.25,0.));
#4554=CARTESIAN_POINT('',(11.5,1.25,0.));
#4555=CARTESIAN_POINT('',(-7.5,1.25,0.6));
#4556=CARTESIAN_POINT('',(-7.5,1.25,0.));
#4557=CARTESIAN_POINT('',(11.5,1.25,0.6));
#4558=CARTESIAN_POINT('',(11.5,1.25,0.6));
#4559=CARTESIAN_POINT('',(11.5,1.25,0.));
#4560=CARTESIAN_POINT('Origin',(11.5,-1.25,0.));
#4561=CARTESIAN_POINT('',(11.5,-1.25,0.));
#4562=CARTESIAN_POINT('',(11.5,-1.25,0.));
#4563=CARTESIAN_POINT('',(11.5,-1.25,0.6));
#4564=CARTESIAN_POINT('',(11.5,-1.25,0.6));
#4565=CARTESIAN_POINT('',(11.5,-1.25,0.));
#4566=CARTESIAN_POINT('Origin',(-7.5,-1.25,0.));
#4567=CARTESIAN_POINT('',(-7.5,-1.25,0.));
#4568=CARTESIAN_POINT('',(-7.5,-1.25,0.));
#4569=CARTESIAN_POINT('',(-7.5,-1.25,0.6));
#4570=CARTESIAN_POINT('',(-7.5,-1.25,0.6));
#4571=CARTESIAN_POINT('',(-7.5,-1.25,0.));
#4572=CARTESIAN_POINT('Origin',(-7.5,1.25,0.));
#4573=CARTESIAN_POINT('',(-7.5,1.25,0.));
#4574=CARTESIAN_POINT('',(-7.5,1.25,0.6));
#4575=CARTESIAN_POINT('Origin',(2.,0.,0.6));
#4576=CARTESIAN_POINT('Origin',(2.,0.,0.));
#5415=UNCERTAINTY_MEASURE_WITH_UNIT(LENGTH_MEASURE(0.001),#5459,
'DISTANCE_ACCURACY_VALUE',
'Maximum model space distance between geometric entities at asserted c
onnectivities');
#5435=UNCERTAINTY_MEASURE_WITH_UNIT(LENGTH_MEASURE(0.001),#5459,
'DISTANCE_ACCURACY_VALUE',
'Maximum model space distance between geometric entities at asserted c
onnectivities');
#5438=(
GEOMETRIC_REPRESENTATION_CONTEXT(3)
GLOBAL_UNCERTAINTY_ASSIGNED_CONTEXT((#5415))
GLOBAL_UNIT_ASSIGNED_CONTEXT((#5459,#5461,#5462))
REPRESENTATION_CONTEXT('','3D')
);
#5458=(
GEOMETRIC_REPRESENTATION_CONTEXT(3)
GLOBAL_UNCERTAINTY_ASSIGNED_CONTEXT((#5435))
GLOBAL_UNIT_ASSIGNED_CONTEXT((#5459,#5461,#5462))
REPRESENTATION_CONTEXT('','3D')
);
#5459=(
LENGTH_UNIT()
NAMED_UNIT(*)
SI_UNIT(.CENTI.,.METRE.)
);
#5461=(
NAMED_UNIT(*)
PLANE_ANGLE_UNIT()
SI_UNIT($,.RADIAN.)
);
#5462=(
NAMED_UNIT(*)
SI_UNIT($,.STERADIAN.)
SOLID_ANGLE_UNIT()
);
#5465=SHAPE_DEFINITION_REPRESENTATION(#5487,#5536);
#5487=PRODUCT_DEFINITION_SHAPE('',$,#5559);
#5536=SHAPE_REPRESENTATION('',(#3178),#5438);
#5556=PRODUCT_DEFINITION_CONTEXT('part definition',#5624,'design');
#5559=PRODUCT_DEFINITION('Pull-toggle base','Pull-toggle base',#5581,#5556);
#5581=PRODUCT_DEFINITION_FORMATION('',$,#5628);
#5624=APPLICATION_CONTEXT(
'Core Data for Automotive Mechanical Design Process');
#5625=PRODUCT_CONTEXT('part definition',#5624,'mechanical');
#5628=PRODUCT('Pull-toggle base','Pull-toggle base','Pull-toggle base',
(#5625));
#5690=COLOUR_RGB('Dark Blue',0.08,0.2,0.34);
#5691=FILL_AREA_STYLE_COLOUR('',#5690);
#5692=FILL_AREA_STYLE('',(#5691));
#5693=SURFACE_STYLE_FILL_AREA(#5692);
#5694=SURFACE_SIDE_STYLE('',(#5693));
#5695=SURFACE_STYLE_USAGE(.BOTH.,#5694);
#5696=PRESENTATION_STYLE_ASSIGNMENT((#5695));
ENDSEC;
END-ISO-10303-21;
